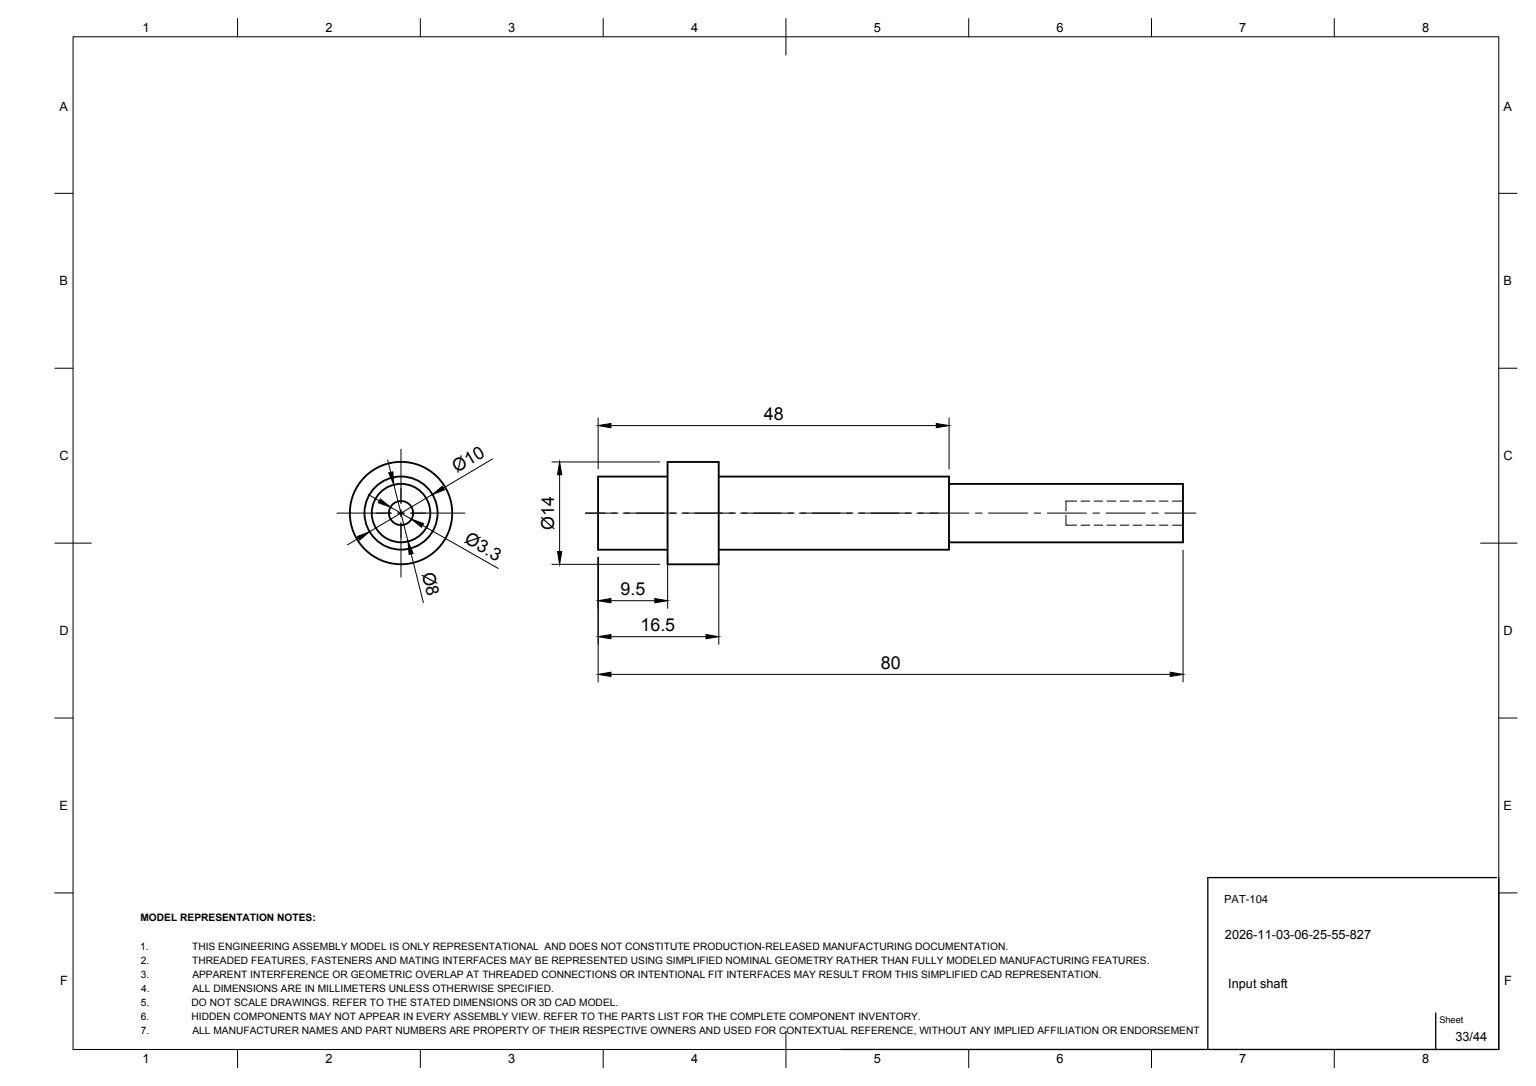
ISO-10303-21;
HEADER;
/* Generated by software containing ST-Developer
 * from STEP Tools, Inc. (www.steptools.com) 
 */

FILE_DESCRIPTION(
/* description */ ('Timing belt drive module 2 mm Pitch Timing 20T-40T'),

/* implementation_level */ '2;1');

FILE_NAME(
/* name */ 'Input shaft.step',
/* time_stamp */ '2026-10-28T03:25:12-07:00',
/* author */ (''),
/* organization */ (''),
/* preprocessor_version */ 'ST-DEVELOPER v20.2',
/* originating_system */ 'Autodesk Translation Framework v15.17.0.0',
/* authorisation */ '');

FILE_SCHEMA (('AUTOMOTIVE_DESIGN { 1 0 10303 214 3 1 1 }'));
ENDSEC;

DATA;
#10=MECHANICAL_DESIGN_GEOMETRIC_PRESENTATION_REPRESENTATION('',(#567),#17830);
#466=SHAPE_REPRESENTATION_RELATIONSHIP('SRR','None',#18039,#509);
#509=ADVANCED_BREP_SHAPE_REPRESENTATION('',(#623),#17814);
#567=STYLED_ITEM('',(#18317),#623);
#623=MANIFOLD_SOLID_BREP('Body1',#9026);
#730=FACE_BOUND('',#1879,.T.);
#731=FACE_BOUND('',#1881,.T.);
#732=FACE_BOUND('',#1886,.T.);
#733=FACE_BOUND('',#1890,.T.);
#909=PLANE('',#10197);
#910=PLANE('',#10198);
#911=PLANE('',#10201);
#912=PLANE('',#10210);
#913=PLANE('',#10213);
#914=PLANE('',#10214);
#1262=FACE_OUTER_BOUND('',#1876,.T.);
#1263=FACE_OUTER_BOUND('',#1877,.T.);
#1264=FACE_OUTER_BOUND('',#1878,.T.);
#1265=FACE_OUTER_BOUND('',#1880,.T.);
#1266=FACE_OUTER_BOUND('',#1882,.T.);
#1267=FACE_OUTER_BOUND('',#1883,.T.);
#1268=FACE_OUTER_BOUND('',#1884,.T.);
#1269=FACE_OUTER_BOUND('',#1885,.T.);
#1270=FACE_OUTER_BOUND('',#1887,.T.);
#1271=FACE_OUTER_BOUND('',#1888,.T.);
#1272=FACE_OUTER_BOUND('',#1889,.T.);
#1876=EDGE_LOOP('',(#7081,#7082,#7083,#7084));
#1877=EDGE_LOOP('',(#7085));
#1878=EDGE_LOOP('',(#7086));
#1879=EDGE_LOOP('',(#7087));
#1880=EDGE_LOOP('',(#7088));
#1881=EDGE_LOOP('',(#7089));
#1882=EDGE_LOOP('',(#7090,#7091,#7092,#7093));
#1883=EDGE_LOOP('',(#7094,#7095,#7096,#7097));
#1884=EDGE_LOOP('',(#7098,#7099,#7100,#7101));
#1885=EDGE_LOOP('',(#7102));
#1886=EDGE_LOOP('',(#7103));
#1887=EDGE_LOOP('',(#7104,#7105,#7106,#7107));
#1888=EDGE_LOOP('',(#7108));
#1889=EDGE_LOOP('',(#7109));
#1890=EDGE_LOOP('',(#7110));
#2474=CIRCLE('',#10195,0.165);
#2475=CIRCLE('',#10196,0.165);
#2476=CIRCLE('',#10199,0.7);
#2477=CIRCLE('',#10200,0.5);
#2478=CIRCLE('',#10202,0.7);
#2479=CIRCLE('',#10203,0.5);
#2480=CIRCLE('',#10206,0.5);
#2481=CIRCLE('',#10208,0.4);
#2482=CIRCLE('',#10209,0.4);
#2483=CIRCLE('',#10212,0.5);
#3078=LINE('',#15958,#3556);
#3079=LINE('',#15972,#3557);
#3080=LINE('',#15975,#3558);
#3081=LINE('',#15981,#3559);
#3082=LINE('',#15987,#3560);
#3556=VECTOR('',#12457,0.165);
#3557=VECTOR('',#12476,0.7);
#3558=VECTOR('',#12479,0.5);
#3559=VECTOR('',#12486,0.4);
#3560=VECTOR('',#12495,0.5);
#4197=VERTEX_POINT('',#15955);
#4198=VERTEX_POINT('',#15957);
#4199=VERTEX_POINT('',#15962);
#4200=VERTEX_POINT('',#15964);
#4201=VERTEX_POINT('',#15967);
#4202=VERTEX_POINT('',#15969);
#4203=VERTEX_POINT('',#15974);
#4204=VERTEX_POINT('',#15978);
#4205=VERTEX_POINT('',#15980);
#4206=VERTEX_POINT('',#15985);
#5223=EDGE_CURVE('',#4197,#4197,#2474,.T.);
#5224=EDGE_CURVE('',#4197,#4198,#3078,.T.);
#5225=EDGE_CURVE('',#4198,#4198,#2475,.T.);
#5226=EDGE_CURVE('',#4199,#4199,#2476,.T.);
#5227=EDGE_CURVE('',#4200,#4200,#2477,.T.);
#5228=EDGE_CURVE('',#4201,#4201,#2478,.T.);
#5229=EDGE_CURVE('',#4202,#4202,#2479,.T.);
#5230=EDGE_CURVE('',#4199,#4201,#3079,.T.);
#5231=EDGE_CURVE('',#4202,#4203,#3080,.T.);
#5232=EDGE_CURVE('',#4203,#4203,#2480,.T.);
#5233=EDGE_CURVE('',#4204,#4204,#2481,.T.);
#5234=EDGE_CURVE('',#4204,#4205,#3081,.T.);
#5235=EDGE_CURVE('',#4205,#4205,#2482,.T.);
#5236=EDGE_CURVE('',#4206,#4206,#2483,.T.);
#5237=EDGE_CURVE('',#4206,#4200,#3082,.T.);
#7081=ORIENTED_EDGE('',*,*,#5223,.F.);
#7082=ORIENTED_EDGE('',*,*,#5224,.T.);
#7083=ORIENTED_EDGE('',*,*,#5225,.T.);
#7084=ORIENTED_EDGE('',*,*,#5224,.F.);
#7085=ORIENTED_EDGE('',*,*,#5225,.F.);
#7086=ORIENTED_EDGE('',*,*,#5226,.T.);
#7087=ORIENTED_EDGE('',*,*,#5227,.F.);
#7088=ORIENTED_EDGE('',*,*,#5228,.F.);
#7089=ORIENTED_EDGE('',*,*,#5229,.F.);
#7090=ORIENTED_EDGE('',*,*,#5226,.F.);
#7091=ORIENTED_EDGE('',*,*,#5230,.T.);
#7092=ORIENTED_EDGE('',*,*,#5228,.T.);
#7093=ORIENTED_EDGE('',*,*,#5230,.F.);
#7094=ORIENTED_EDGE('',*,*,#5229,.T.);
#7095=ORIENTED_EDGE('',*,*,#5231,.T.);
#7096=ORIENTED_EDGE('',*,*,#5232,.T.);
#7097=ORIENTED_EDGE('',*,*,#5231,.F.);
#7098=ORIENTED_EDGE('',*,*,#5233,.F.);
#7099=ORIENTED_EDGE('',*,*,#5234,.T.);
#7100=ORIENTED_EDGE('',*,*,#5235,.T.);
#7101=ORIENTED_EDGE('',*,*,#5234,.F.);
#7102=ORIENTED_EDGE('',*,*,#5235,.F.);
#7103=ORIENTED_EDGE('',*,*,#5223,.T.);
#7104=ORIENTED_EDGE('',*,*,#5236,.F.);
#7105=ORIENTED_EDGE('',*,*,#5237,.T.);
#7106=ORIENTED_EDGE('',*,*,#5227,.T.);
#7107=ORIENTED_EDGE('',*,*,#5237,.F.);
#7108=ORIENTED_EDGE('',*,*,#5236,.T.);
#7109=ORIENTED_EDGE('',*,*,#5232,.F.);
#7110=ORIENTED_EDGE('',*,*,#5233,.T.);
#8296=CYLINDRICAL_SURFACE('',#10194,0.165);
#8297=CYLINDRICAL_SURFACE('',#10204,0.7);
#8298=CYLINDRICAL_SURFACE('',#10205,0.5);
#8299=CYLINDRICAL_SURFACE('',#10207,0.4);
#8300=CYLINDRICAL_SURFACE('',#10211,0.5);
#8760=ADVANCED_FACE('',(#1262),#8296,.F.);
#8761=ADVANCED_FACE('',(#1263),#909,.F.);
#8762=ADVANCED_FACE('',(#1264,#730),#910,.T.);
#8763=ADVANCED_FACE('',(#1265,#731),#911,.F.);
#8764=ADVANCED_FACE('',(#1266),#8297,.T.);
#8765=ADVANCED_FACE('',(#1267),#8298,.T.);
#8766=ADVANCED_FACE('',(#1268),#8299,.T.);
#8767=ADVANCED_FACE('',(#1269,#732),#912,.F.);
#8768=ADVANCED_FACE('',(#1270),#8300,.T.);
#8769=ADVANCED_FACE('',(#1271),#913,.T.);
#8770=ADVANCED_FACE('',(#1272,#733),#914,.F.);
#9026=CLOSED_SHELL('',(#8760,#8761,#8762,#8763,#8764,#8765,#8766,#8767,
#8768,#8769,#8770));
#10193=AXIS2_PLACEMENT_3D('',#15953,#12451,#12452);
#10194=AXIS2_PLACEMENT_3D('',#15954,#12453,#12454);
#10195=AXIS2_PLACEMENT_3D('',#15956,#12455,#12456);
#10196=AXIS2_PLACEMENT_3D('',#15959,#12458,#12459);
#10197=AXIS2_PLACEMENT_3D('',#15960,#12460,#12461);
#10198=AXIS2_PLACEMENT_3D('',#15961,#12462,#12463);
#10199=AXIS2_PLACEMENT_3D('',#15963,#12464,#12465);
#10200=AXIS2_PLACEMENT_3D('',#15965,#12466,#12467);
#10201=AXIS2_PLACEMENT_3D('',#15966,#12468,#12469);
#10202=AXIS2_PLACEMENT_3D('',#15968,#12470,#12471);
#10203=AXIS2_PLACEMENT_3D('',#15970,#12472,#12473);
#10204=AXIS2_PLACEMENT_3D('',#15971,#12474,#12475);
#10205=AXIS2_PLACEMENT_3D('',#15973,#12477,#12478);
#10206=AXIS2_PLACEMENT_3D('',#15976,#12480,#12481);
#10207=AXIS2_PLACEMENT_3D('',#15977,#12482,#12483);
#10208=AXIS2_PLACEMENT_3D('',#15979,#12484,#12485);
#10209=AXIS2_PLACEMENT_3D('',#15982,#12487,#12488);
#10210=AXIS2_PLACEMENT_3D('',#15983,#12489,#12490);
#10211=AXIS2_PLACEMENT_3D('',#15984,#12491,#12492);
#10212=AXIS2_PLACEMENT_3D('',#15986,#12493,#12494);
#10213=AXIS2_PLACEMENT_3D('',#15988,#12496,#12497);
#10214=AXIS2_PLACEMENT_3D('',#15989,#12498,#12499);
#12451=DIRECTION('axis',(0.,0.,1.));
#12452=DIRECTION('refdir',(1.,0.,0.));
#12453=DIRECTION('center_axis',(0.,1.,0.));
#12454=DIRECTION('ref_axis',(1.,0.,0.));
#12455=DIRECTION('center_axis',(0.,1.,0.));
#12456=DIRECTION('ref_axis',(1.,0.,0.));
#12457=DIRECTION('',(0.,1.,0.));
#12458=DIRECTION('center_axis',(0.,1.,0.));
#12459=DIRECTION('ref_axis',(1.,0.,0.));
#12460=DIRECTION('center_axis',(0.,1.,0.));
#12461=DIRECTION('ref_axis',(1.,0.,0.));
#12462=DIRECTION('center_axis',(0.,1.,0.));
#12463=DIRECTION('ref_axis',(1.,0.,0.));
#12464=DIRECTION('center_axis',(0.,1.,0.));
#12465=DIRECTION('ref_axis',(1.,0.,0.));
#12466=DIRECTION('center_axis',(0.,1.,0.));
#12467=DIRECTION('ref_axis',(1.,0.,0.));
#12468=DIRECTION('center_axis',(0.,1.,0.));
#12469=DIRECTION('ref_axis',(1.,0.,0.));
#12470=DIRECTION('center_axis',(0.,1.,0.));
#12471=DIRECTION('ref_axis',(1.,0.,0.));
#12472=DIRECTION('center_axis',(0.,-1.,0.));
#12473=DIRECTION('ref_axis',(1.,0.,0.));
#12474=DIRECTION('center_axis',(0.,1.,0.));
#12475=DIRECTION('ref_axis',(1.,0.,0.));
#12476=DIRECTION('',(0.,-1.,0.));
#12477=DIRECTION('center_axis',(0.,1.,0.));
#12478=DIRECTION('ref_axis',(1.,0.,0.));
#12479=DIRECTION('',(0.,-1.,0.));
#12480=DIRECTION('center_axis',(0.,1.,0.));
#12481=DIRECTION('ref_axis',(1.,0.,0.));
#12482=DIRECTION('center_axis',(0.,1.,0.));
#12483=DIRECTION('ref_axis',(1.,0.,0.));
#12484=DIRECTION('center_axis',(0.,1.,0.));
#12485=DIRECTION('ref_axis',(1.,0.,0.));
#12486=DIRECTION('',(0.,-1.,0.));
#12487=DIRECTION('center_axis',(0.,1.,0.));
#12488=DIRECTION('ref_axis',(1.,0.,0.));
#12489=DIRECTION('center_axis',(0.,1.,0.));
#12490=DIRECTION('ref_axis',(1.,0.,0.));
#12491=DIRECTION('center_axis',(0.,1.,0.));
#12492=DIRECTION('ref_axis',(1.,0.,0.));
#12493=DIRECTION('center_axis',(0.,1.,0.));
#12494=DIRECTION('ref_axis',(1.,0.,0.));
#12495=DIRECTION('',(0.,-1.,0.));
#12496=DIRECTION('center_axis',(0.,1.,0.));
#12497=DIRECTION('ref_axis',(1.,0.,0.));
#12498=DIRECTION('center_axis',(0.,1.,0.));
#12499=DIRECTION('ref_axis',(1.,0.,0.));
#15953=CARTESIAN_POINT('',(0.,0.,0.));
#15954=CARTESIAN_POINT('Origin',(0.,-5.1,7.));
#15955=CARTESIAN_POINT('',(-0.165,-5.,7.));
#15956=CARTESIAN_POINT('Origin',(0.,-5.,7.));
#15957=CARTESIAN_POINT('',(-0.165,-3.4,7.));
#15958=CARTESIAN_POINT('',(-0.165,-5.1,7.));
#15959=CARTESIAN_POINT('Origin',(0.,-3.4,7.));
#15960=CARTESIAN_POINT('Origin',(0.,-3.4,7.));
#15961=CARTESIAN_POINT('Origin',(0.,2.05,7.));
#15962=CARTESIAN_POINT('',(-0.7,2.05,7.));
#15963=CARTESIAN_POINT('Origin',(0.,2.05,7.));
#15964=CARTESIAN_POINT('',(-0.5,2.05,7.));
#15965=CARTESIAN_POINT('Origin',(0.,2.05,7.));
#15966=CARTESIAN_POINT('Origin',(0.,1.35,7.));
#15967=CARTESIAN_POINT('',(-0.7,1.35,7.));
#15968=CARTESIAN_POINT('Origin',(0.,1.35,7.));
#15969=CARTESIAN_POINT('',(-0.5,1.35,7.));
#15970=CARTESIAN_POINT('Origin',(0.,1.35,7.));
#15971=CARTESIAN_POINT('Origin',(0.,1.35,7.));
#15972=CARTESIAN_POINT('',(-0.7,1.35,7.));
#15973=CARTESIAN_POINT('Origin',(0.,-1.8,7.));
#15974=CARTESIAN_POINT('',(-0.5,-1.8,7.));
#15975=CARTESIAN_POINT('',(-0.5,-1.8,7.));
#15976=CARTESIAN_POINT('Origin',(0.,-1.8,7.));
#15977=CARTESIAN_POINT('Origin',(0.,-5.,7.));
#15978=CARTESIAN_POINT('',(-0.4,-1.8,7.));
#15979=CARTESIAN_POINT('Origin',(0.,-1.8,7.));
#15980=CARTESIAN_POINT('',(-0.4,-5.,7.));
#15981=CARTESIAN_POINT('',(-0.4,-5.,7.));
#15982=CARTESIAN_POINT('Origin',(0.,-5.,7.));
#15983=CARTESIAN_POINT('Origin',(0.,-5.,7.));
#15984=CARTESIAN_POINT('Origin',(0.,-1.8,7.));
#15985=CARTESIAN_POINT('',(-0.5,3.,7.));
#15986=CARTESIAN_POINT('Origin',(0.,3.,7.));
#15987=CARTESIAN_POINT('',(-0.5,-1.8,7.));
#15988=CARTESIAN_POINT('Origin',(0.,3.,7.));
#15989=CARTESIAN_POINT('Origin',(0.,-1.8,7.));
#17764=UNCERTAINTY_MEASURE_WITH_UNIT(LENGTH_MEASURE(0.001),#17831,
'DISTANCE_ACCURACY_VALUE',
'Maximum model space distance between geometric entities at asserted c
onnectivities');
#17780=UNCERTAINTY_MEASURE_WITH_UNIT(LENGTH_MEASURE(0.001),#17831,
'DISTANCE_ACCURACY_VALUE',
'Maximum model space distance between geometric entities at asserted c
onnectivities');
#17814=(
GEOMETRIC_REPRESENTATION_CONTEXT(3)
GLOBAL_UNCERTAINTY_ASSIGNED_CONTEXT((#17764))
GLOBAL_UNIT_ASSIGNED_CONTEXT((#17831,#17833,#17834))
REPRESENTATION_CONTEXT('','3D')
);
#17830=(
GEOMETRIC_REPRESENTATION_CONTEXT(3)
GLOBAL_UNCERTAINTY_ASSIGNED_CONTEXT((#17780))
GLOBAL_UNIT_ASSIGNED_CONTEXT((#17831,#17833,#17834))
REPRESENTATION_CONTEXT('','3D')
);
#17831=(
LENGTH_UNIT()
NAMED_UNIT(*)
SI_UNIT(.CENTI.,.METRE.)
);
#17833=(
NAMED_UNIT(*)
PLANE_ANGLE_UNIT()
SI_UNIT($,.RADIAN.)
);
#17834=(
NAMED_UNIT(*)
SI_UNIT($,.STERADIAN.)
SOLID_ANGLE_UNIT()
);
#17868=SHAPE_DEFINITION_REPRESENTATION(#17927,#18039);
#17927=PRODUCT_DEFINITION_SHAPE('',$,#18089);
#18039=SHAPE_REPRESENTATION('',(#10193),#17814);
#18055=PRODUCT_DEFINITION_CONTEXT('part definition',#18204,'design');
#18089=PRODUCT_DEFINITION('Input shaft','Input shaft',#18138,#18055);
#18138=PRODUCT_DEFINITION_FORMATION('',$,#18239);
#18204=APPLICATION_CONTEXT(
'Core Data for Automotive Mechanical Design Process');
#18205=PRODUCT_CONTEXT('part definition',#18204,'mechanical');
#18239=PRODUCT('Input shaft','Input shaft','Input shaft',(#18205));
#18311=COLOUR_RGB('Grey',0.48,0.52,0.57);
#18312=FILL_AREA_STYLE_COLOUR('',#18311);
#18313=FILL_AREA_STYLE('',(#18312));
#18314=SURFACE_STYLE_FILL_AREA(#18313);
#18315=SURFACE_SIDE_STYLE('',(#18314));
#18316=SURFACE_STYLE_USAGE(.BOTH.,#18315);
#18317=PRESENTATION_STYLE_ASSIGNMENT((#18316));
ENDSEC;
END-ISO-10303-21;
